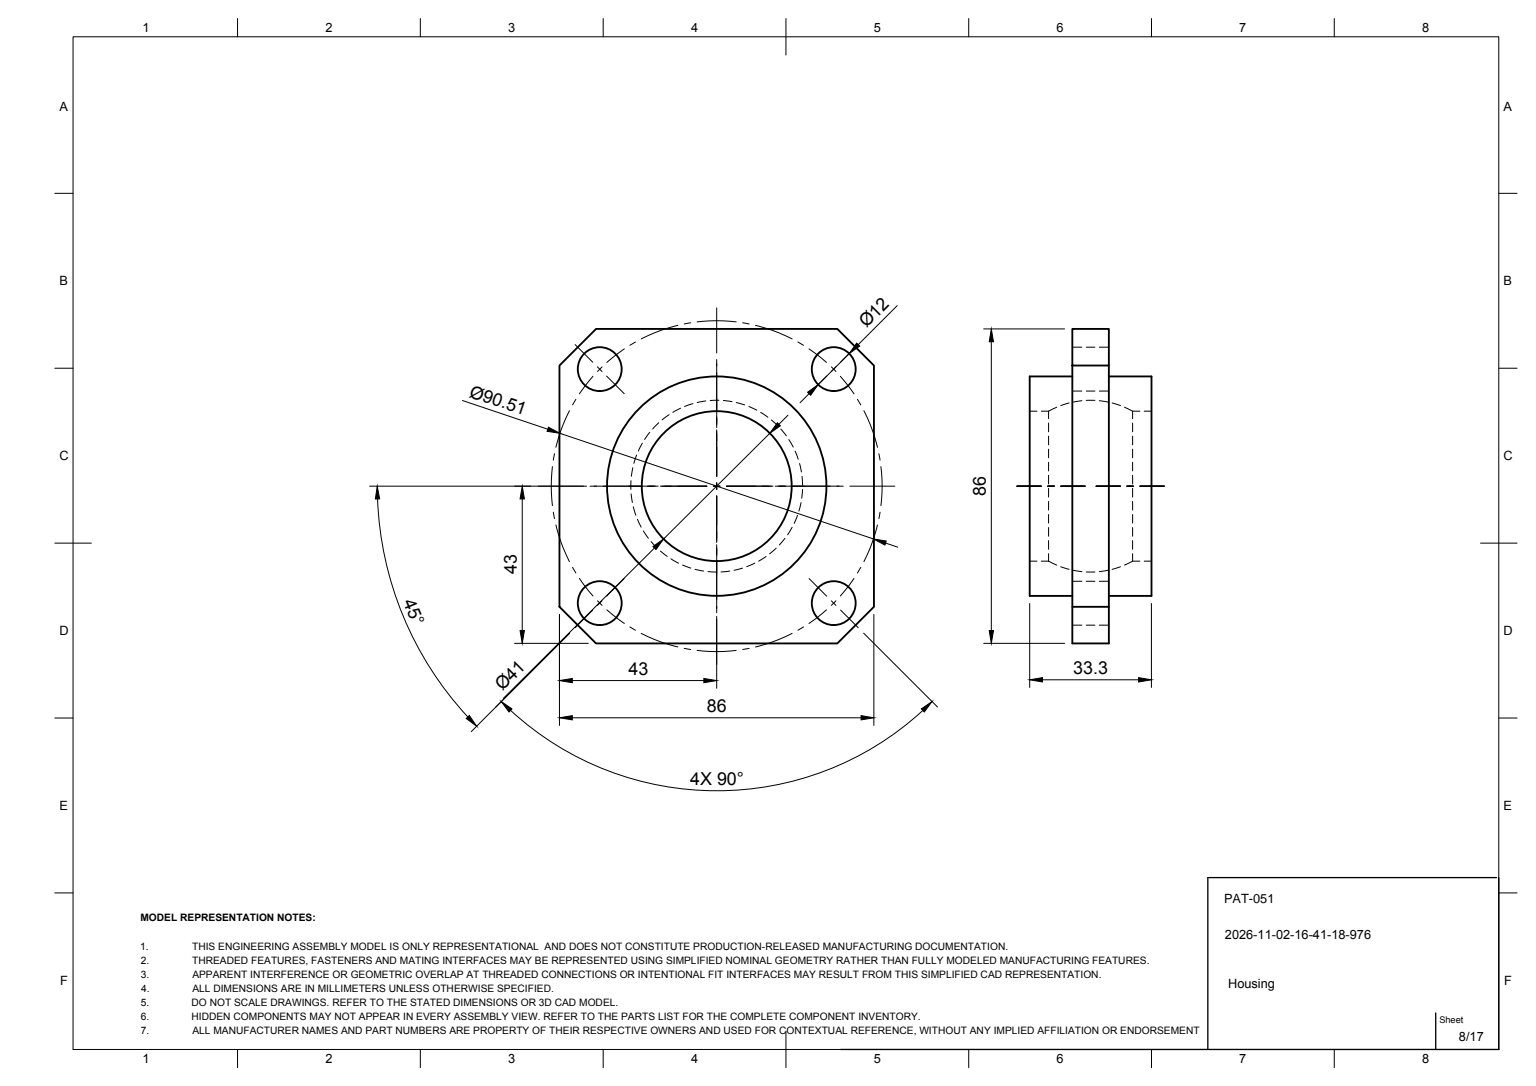
ISO-10303-21;
HEADER;
/* Generated by software containing ST-Developer
 * from STEP Tools, Inc. (www.steptools.com) 
 */

FILE_DESCRIPTION(
/* description */ ('Hand-crank flanged shaft unit'),
/* implementation_level */ '2;1');

FILE_NAME(
/* name */ 'Housing.step',
/* time_stamp */ '2026-10-27T18:35:45-07:00',
/* author */ (''),
/* organization */ (''),
/* preprocessor_version */ 'ST-DEVELOPER v20.2',
/* originating_system */ 'Autodesk Translation Framework v15.17.0.0',
/* authorisation */ '');

FILE_SCHEMA (('AUTOMOTIVE_DESIGN { 1 0 10303 214 3 1 1 }'));
ENDSEC;

DATA;
#10=MECHANICAL_DESIGN_GEOMETRIC_PRESENTATION_REPRESENTATION('',(#288),#6805);
#237=SPHERICAL_SURFACE('',#3681,2.35);
#248=SHAPE_REPRESENTATION_RELATIONSHIP('SRR','None',#6910,#268);
#268=ADVANCED_BREP_SHAPE_REPRESENTATION('',(#309),#6793);
#288=STYLED_ITEM('',(#7070),#309);
#309=MANIFOLD_SOLID_BREP('Body1',#3329);
#358=FACE_BOUND('',#802,.T.);
#359=FACE_BOUND('',#803,.T.);
#360=FACE_BOUND('',#807,.T.);
#361=FACE_BOUND('',#809,.T.);
#362=FACE_BOUND('',#823,.T.);
#363=FACE_BOUND('',#824,.T.);
#364=FACE_BOUND('',#825,.T.);
#365=FACE_BOUND('',#826,.T.);
#366=FACE_BOUND('',#827,.T.);
#367=FACE_BOUND('',#829,.T.);
#368=FACE_BOUND('',#830,.T.);
#369=FACE_BOUND('',#831,.T.);
#370=FACE_BOUND('',#832,.T.);
#371=FACE_BOUND('',#833,.T.);
#442=PLANE('',#3689);
#443=PLANE('',#3690);
#444=PLANE('',#3703);
#445=PLANE('',#3704);
#446=PLANE('',#3705);
#447=PLANE('',#3706);
#448=PLANE('',#3707);
#449=PLANE('',#3708);
#450=PLANE('',#3709);
#451=PLANE('',#3710);
#452=PLANE('',#3711);
#453=PLANE('',#3712);
#573=FACE_OUTER_BOUND('',#799,.T.);
#574=FACE_OUTER_BOUND('',#800,.T.);
#575=FACE_OUTER_BOUND('',#801,.T.);
#576=FACE_OUTER_BOUND('',#804,.T.);
#577=FACE_OUTER_BOUND('',#805,.T.);
#578=FACE_OUTER_BOUND('',#806,.T.);
#579=FACE_OUTER_BOUND('',#808,.T.);
#580=FACE_OUTER_BOUND('',#810,.T.);
#581=FACE_OUTER_BOUND('',#811,.T.);
#582=FACE_OUTER_BOUND('',#812,.T.);
#583=FACE_OUTER_BOUND('',#813,.T.);
#584=FACE_OUTER_BOUND('',#814,.T.);
#585=FACE_OUTER_BOUND('',#815,.T.);
#586=FACE_OUTER_BOUND('',#816,.T.);
#587=FACE_OUTER_BOUND('',#817,.T.);
#588=FACE_OUTER_BOUND('',#818,.T.);
#589=FACE_OUTER_BOUND('',#819,.T.);
#590=FACE_OUTER_BOUND('',#820,.T.);
#591=FACE_OUTER_BOUND('',#821,.T.);
#592=FACE_OUTER_BOUND('',#822,.T.);
#593=FACE_OUTER_BOUND('',#828,.T.);
#799=EDGE_LOOP('',(#2479,#2480,#2481,#2482));
#800=EDGE_LOOP('',(#2483,#2484,#2485,#2486));
#801=EDGE_LOOP('',(#2487,#2488));
#802=EDGE_LOOP('',(#2489));
#803=EDGE_LOOP('',(#2490));
#804=EDGE_LOOP('',(#2491,#2492,#2493,#2494));
#805=EDGE_LOOP('',(#2495,#2496,#2497,#2498));
#806=EDGE_LOOP('',(#2499));
#807=EDGE_LOOP('',(#2500));
#808=EDGE_LOOP('',(#2501));
#809=EDGE_LOOP('',(#2502));
#810=EDGE_LOOP('',(#2503,#2504,#2505,#2506));
#811=EDGE_LOOP('',(#2507,#2508,#2509,#2510));
#812=EDGE_LOOP('',(#2511,#2512,#2513,#2514));
#813=EDGE_LOOP('',(#2515,#2516,#2517,#2518));
#814=EDGE_LOOP('',(#2519,#2520,#2521,#2522));
#815=EDGE_LOOP('',(#2523,#2524,#2525,#2526));
#816=EDGE_LOOP('',(#2527,#2528,#2529,#2530));
#817=EDGE_LOOP('',(#2531,#2532,#2533,#2534));
#818=EDGE_LOOP('',(#2535,#2536,#2537,#2538));
#819=EDGE_LOOP('',(#2539,#2540,#2541,#2542));
#820=EDGE_LOOP('',(#2543,#2544,#2545,#2546));
#821=EDGE_LOOP('',(#2547,#2548,#2549,#2550));
#822=EDGE_LOOP('',(#2551,#2552,#2553,#2554,#2555,#2556,#2557,#2558));
#823=EDGE_LOOP('',(#2559));
#824=EDGE_LOOP('',(#2560));
#825=EDGE_LOOP('',(#2561));
#826=EDGE_LOOP('',(#2562));
#827=EDGE_LOOP('',(#2563));
#828=EDGE_LOOP('',(#2564,#2565,#2566,#2567,#2568,#2569,#2570,#2571));
#829=EDGE_LOOP('',(#2572));
#830=EDGE_LOOP('',(#2573));
#831=EDGE_LOOP('',(#2574));
#832=EDGE_LOOP('',(#2575));
#833=EDGE_LOOP('',(#2576));
#1043=LINE('',#5197,#1271);
#1044=LINE('',#5203,#1272);
#1045=LINE('',#5213,#1273);
#1046=LINE('',#5219,#1274);
#1047=LINE('',#5227,#1275);
#1048=LINE('',#5233,#1276);
#1049=LINE('',#5239,#1277);
#1050=LINE('',#5245,#1278);
#1051=LINE('',#5250,#1279);
#1052=LINE('',#5252,#1280);
#1053=LINE('',#5254,#1281);
#1054=LINE('',#5255,#1282);
#1055=LINE('',#5258,#1283);
#1056=LINE('',#5260,#1284);
#1057=LINE('',#5261,#1285);
#1058=LINE('',#5264,#1286);
#1059=LINE('',#5266,#1287);
#1060=LINE('',#5267,#1288);
#1061=LINE('',#5270,#1289);
#1062=LINE('',#5272,#1290);
#1063=LINE('',#5273,#1291);
#1064=LINE('',#5276,#1292);
#1065=LINE('',#5278,#1293);
#1066=LINE('',#5279,#1294);
#1067=LINE('',#5282,#1295);
#1068=LINE('',#5284,#1296);
#1069=LINE('',#5285,#1297);
#1070=LINE('',#5288,#1298);
#1071=LINE('',#5290,#1299);
#1072=LINE('',#5291,#1300);
#1073=LINE('',#5293,#1301);
#1074=LINE('',#5294,#1302);
#1271=VECTOR('',#4248,2.05);
#1272=VECTOR('',#4255,2.05);
#1273=VECTOR('',#4266,3.);
#1274=VECTOR('',#4273,3.);
#1275=VECTOR('',#4284,0.6);
#1276=VECTOR('',#4291,0.6);
#1277=VECTOR('',#4298,0.6);
#1278=VECTOR('',#4305,0.6);
#1279=VECTOR('',#4310,1.);
#1280=VECTOR('',#4311,1.);
#1281=VECTOR('',#4312,1.);
#1282=VECTOR('',#4313,1.);
#1283=VECTOR('',#4316,1.);
#1284=VECTOR('',#4317,1.);
#1285=VECTOR('',#4318,1.);
#1286=VECTOR('',#4321,1.);
#1287=VECTOR('',#4322,1.);
#1288=VECTOR('',#4323,1.);
#1289=VECTOR('',#4326,1.);
#1290=VECTOR('',#4327,1.);
#1291=VECTOR('',#4328,1.);
#1292=VECTOR('',#4331,1.);
#1293=VECTOR('',#4332,1.);
#1294=VECTOR('',#4333,1.);
#1295=VECTOR('',#4336,1.);
#1296=VECTOR('',#4337,1.);
#1297=VECTOR('',#4338,1.);
#1298=VECTOR('',#4341,1.);
#1299=VECTOR('',#4342,1.);
#1300=VECTOR('',#4343,1.);
#1301=VECTOR('',#4346,1.);
#1302=VECTOR('',#4347,1.);
#1489=CIRCLE('',#3676,2.05);
#1490=CIRCLE('',#3677,2.05);
#1491=CIRCLE('',#3679,2.05);
#1492=CIRCLE('',#3680,2.05);
#1493=CIRCLE('',#3682,2.35);
#1494=CIRCLE('',#3684,3.);
#1495=CIRCLE('',#3685,3.);
#1496=CIRCLE('',#3687,3.);
#1497=CIRCLE('',#3688,3.);
#1498=CIRCLE('',#3692,0.6);
#1499=CIRCLE('',#3693,0.6);
#1500=CIRCLE('',#3695,0.6);
#1501=CIRCLE('',#3696,0.6);
#1502=CIRCLE('',#3698,0.6);
#1503=CIRCLE('',#3699,0.6);
#1504=CIRCLE('',#3701,0.6);
#1505=CIRCLE('',#3702,0.6);
#1645=VERTEX_POINT('',#5194);
#1646=VERTEX_POINT('',#5196);
#1647=VERTEX_POINT('',#5200);
#1648=VERTEX_POINT('',#5202);
#1649=VERTEX_POINT('',#5206);
#1650=VERTEX_POINT('',#5207);
#1651=VERTEX_POINT('',#5210);
#1652=VERTEX_POINT('',#5212);
#1653=VERTEX_POINT('',#5216);
#1654=VERTEX_POINT('',#5218);
#1655=VERTEX_POINT('',#5224);
#1656=VERTEX_POINT('',#5226);
#1657=VERTEX_POINT('',#5230);
#1658=VERTEX_POINT('',#5232);
#1659=VERTEX_POINT('',#5236);
#1660=VERTEX_POINT('',#5238);
#1661=VERTEX_POINT('',#5242);
#1662=VERTEX_POINT('',#5244);
#1663=VERTEX_POINT('',#5248);
#1664=VERTEX_POINT('',#5249);
#1665=VERTEX_POINT('',#5251);
#1666=VERTEX_POINT('',#5253);
#1667=VERTEX_POINT('',#5257);
#1668=VERTEX_POINT('',#5259);
#1669=VERTEX_POINT('',#5263);
#1670=VERTEX_POINT('',#5265);
#1671=VERTEX_POINT('',#5269);
#1672=VERTEX_POINT('',#5271);
#1673=VERTEX_POINT('',#5275);
#1674=VERTEX_POINT('',#5277);
#1675=VERTEX_POINT('',#5281);
#1676=VERTEX_POINT('',#5283);
#1677=VERTEX_POINT('',#5287);
#1678=VERTEX_POINT('',#5289);
#1957=EDGE_CURVE('',#1645,#1645,#1489,.T.);
#1958=EDGE_CURVE('',#1645,#1646,#1043,.T.);
#1959=EDGE_CURVE('',#1646,#1646,#1490,.T.);
#1960=EDGE_CURVE('',#1647,#1647,#1491,.T.);
#1961=EDGE_CURVE('',#1647,#1648,#1044,.T.);
#1962=EDGE_CURVE('',#1648,#1648,#1492,.T.);
#1963=EDGE_CURVE('',#1649,#1650,#1493,.T.);
#1964=EDGE_CURVE('',#1651,#1651,#1494,.T.);
#1965=EDGE_CURVE('',#1651,#1652,#1045,.T.);
#1966=EDGE_CURVE('',#1652,#1652,#1495,.T.);
#1967=EDGE_CURVE('',#1653,#1653,#1496,.T.);
#1968=EDGE_CURVE('',#1653,#1654,#1046,.T.);
#1969=EDGE_CURVE('',#1654,#1654,#1497,.T.);
#1970=EDGE_CURVE('',#1655,#1655,#1498,.T.);
#1971=EDGE_CURVE('',#1655,#1656,#1047,.T.);
#1972=EDGE_CURVE('',#1656,#1656,#1499,.T.);
#1973=EDGE_CURVE('',#1657,#1657,#1500,.T.);
#1974=EDGE_CURVE('',#1657,#1658,#1048,.T.);
#1975=EDGE_CURVE('',#1658,#1658,#1501,.T.);
#1976=EDGE_CURVE('',#1659,#1659,#1502,.T.);
#1977=EDGE_CURVE('',#1659,#1660,#1049,.T.);
#1978=EDGE_CURVE('',#1660,#1660,#1503,.T.);
#1979=EDGE_CURVE('',#1661,#1661,#1504,.T.);
#1980=EDGE_CURVE('',#1661,#1662,#1050,.T.);
#1981=EDGE_CURVE('',#1662,#1662,#1505,.T.);
#1982=EDGE_CURVE('',#1663,#1664,#1051,.T.);
#1983=EDGE_CURVE('',#1664,#1665,#1052,.T.);
#1984=EDGE_CURVE('',#1666,#1665,#1053,.T.);
#1985=EDGE_CURVE('',#1663,#1666,#1054,.T.);
#1986=EDGE_CURVE('',#1667,#1663,#1055,.T.);
#1987=EDGE_CURVE('',#1668,#1666,#1056,.T.);
#1988=EDGE_CURVE('',#1667,#1668,#1057,.T.);
#1989=EDGE_CURVE('',#1669,#1667,#1058,.T.);
#1990=EDGE_CURVE('',#1670,#1668,#1059,.T.);
#1991=EDGE_CURVE('',#1669,#1670,#1060,.T.);
#1992=EDGE_CURVE('',#1671,#1669,#1061,.T.);
#1993=EDGE_CURVE('',#1672,#1670,#1062,.T.);
#1994=EDGE_CURVE('',#1671,#1672,#1063,.T.);
#1995=EDGE_CURVE('',#1673,#1671,#1064,.T.);
#1996=EDGE_CURVE('',#1674,#1672,#1065,.T.);
#1997=EDGE_CURVE('',#1673,#1674,#1066,.T.);
#1998=EDGE_CURVE('',#1675,#1673,#1067,.T.);
#1999=EDGE_CURVE('',#1676,#1674,#1068,.T.);
#2000=EDGE_CURVE('',#1675,#1676,#1069,.T.);
#2001=EDGE_CURVE('',#1677,#1675,#1070,.T.);
#2002=EDGE_CURVE('',#1678,#1676,#1071,.T.);
#2003=EDGE_CURVE('',#1677,#1678,#1072,.T.);
#2004=EDGE_CURVE('',#1664,#1677,#1073,.T.);
#2005=EDGE_CURVE('',#1665,#1678,#1074,.T.);
#2479=ORIENTED_EDGE('',*,*,#1957,.F.);
#2480=ORIENTED_EDGE('',*,*,#1958,.T.);
#2481=ORIENTED_EDGE('',*,*,#1959,.F.);
#2482=ORIENTED_EDGE('',*,*,#1958,.F.);
#2483=ORIENTED_EDGE('',*,*,#1960,.F.);
#2484=ORIENTED_EDGE('',*,*,#1961,.T.);
#2485=ORIENTED_EDGE('',*,*,#1962,.F.);
#2486=ORIENTED_EDGE('',*,*,#1961,.F.);
#2487=ORIENTED_EDGE('',*,*,#1963,.T.);
#2488=ORIENTED_EDGE('',*,*,#1963,.F.);
#2489=ORIENTED_EDGE('',*,*,#1960,.T.);
#2490=ORIENTED_EDGE('',*,*,#1959,.T.);
#2491=ORIENTED_EDGE('',*,*,#1964,.F.);
#2492=ORIENTED_EDGE('',*,*,#1965,.T.);
#2493=ORIENTED_EDGE('',*,*,#1966,.F.);
#2494=ORIENTED_EDGE('',*,*,#1965,.F.);
#2495=ORIENTED_EDGE('',*,*,#1967,.F.);
#2496=ORIENTED_EDGE('',*,*,#1968,.T.);
#2497=ORIENTED_EDGE('',*,*,#1969,.F.);
#2498=ORIENTED_EDGE('',*,*,#1968,.F.);
#2499=ORIENTED_EDGE('',*,*,#1966,.T.);
#2500=ORIENTED_EDGE('',*,*,#1957,.T.);
#2501=ORIENTED_EDGE('',*,*,#1967,.T.);
#2502=ORIENTED_EDGE('',*,*,#1962,.T.);
#2503=ORIENTED_EDGE('',*,*,#1970,.F.);
#2504=ORIENTED_EDGE('',*,*,#1971,.T.);
#2505=ORIENTED_EDGE('',*,*,#1972,.F.);
#2506=ORIENTED_EDGE('',*,*,#1971,.F.);
#2507=ORIENTED_EDGE('',*,*,#1973,.F.);
#2508=ORIENTED_EDGE('',*,*,#1974,.T.);
#2509=ORIENTED_EDGE('',*,*,#1975,.F.);
#2510=ORIENTED_EDGE('',*,*,#1974,.F.);
#2511=ORIENTED_EDGE('',*,*,#1976,.F.);
#2512=ORIENTED_EDGE('',*,*,#1977,.T.);
#2513=ORIENTED_EDGE('',*,*,#1978,.F.);
#2514=ORIENTED_EDGE('',*,*,#1977,.F.);
#2515=ORIENTED_EDGE('',*,*,#1979,.F.);
#2516=ORIENTED_EDGE('',*,*,#1980,.T.);
#2517=ORIENTED_EDGE('',*,*,#1981,.F.);
#2518=ORIENTED_EDGE('',*,*,#1980,.F.);
#2519=ORIENTED_EDGE('',*,*,#1982,.T.);
#2520=ORIENTED_EDGE('',*,*,#1983,.T.);
#2521=ORIENTED_EDGE('',*,*,#1984,.F.);
#2522=ORIENTED_EDGE('',*,*,#1985,.F.);
#2523=ORIENTED_EDGE('',*,*,#1986,.T.);
#2524=ORIENTED_EDGE('',*,*,#1985,.T.);
#2525=ORIENTED_EDGE('',*,*,#1987,.F.);
#2526=ORIENTED_EDGE('',*,*,#1988,.F.);
#2527=ORIENTED_EDGE('',*,*,#1989,.T.);
#2528=ORIENTED_EDGE('',*,*,#1988,.T.);
#2529=ORIENTED_EDGE('',*,*,#1990,.F.);
#2530=ORIENTED_EDGE('',*,*,#1991,.F.);
#2531=ORIENTED_EDGE('',*,*,#1992,.T.);
#2532=ORIENTED_EDGE('',*,*,#1991,.T.);
#2533=ORIENTED_EDGE('',*,*,#1993,.F.);
#2534=ORIENTED_EDGE('',*,*,#1994,.F.);
#2535=ORIENTED_EDGE('',*,*,#1995,.T.);
#2536=ORIENTED_EDGE('',*,*,#1994,.T.);
#2537=ORIENTED_EDGE('',*,*,#1996,.F.);
#2538=ORIENTED_EDGE('',*,*,#1997,.F.);
#2539=ORIENTED_EDGE('',*,*,#1998,.T.);
#2540=ORIENTED_EDGE('',*,*,#1997,.T.);
#2541=ORIENTED_EDGE('',*,*,#1999,.F.);
#2542=ORIENTED_EDGE('',*,*,#2000,.F.);
#2543=ORIENTED_EDGE('',*,*,#2001,.T.);
#2544=ORIENTED_EDGE('',*,*,#2000,.T.);
#2545=ORIENTED_EDGE('',*,*,#2002,.F.);
#2546=ORIENTED_EDGE('',*,*,#2003,.F.);
#2547=ORIENTED_EDGE('',*,*,#2004,.T.);
#2548=ORIENTED_EDGE('',*,*,#2003,.T.);
#2549=ORIENTED_EDGE('',*,*,#2005,.F.);
#2550=ORIENTED_EDGE('',*,*,#1983,.F.);
#2551=ORIENTED_EDGE('',*,*,#2005,.T.);
#2552=ORIENTED_EDGE('',*,*,#2002,.T.);
#2553=ORIENTED_EDGE('',*,*,#1999,.T.);
#2554=ORIENTED_EDGE('',*,*,#1996,.T.);
#2555=ORIENTED_EDGE('',*,*,#1993,.T.);
#2556=ORIENTED_EDGE('',*,*,#1990,.T.);
#2557=ORIENTED_EDGE('',*,*,#1987,.T.);
#2558=ORIENTED_EDGE('',*,*,#1984,.T.);
#2559=ORIENTED_EDGE('',*,*,#1969,.T.);
#2560=ORIENTED_EDGE('',*,*,#1972,.T.);
#2561=ORIENTED_EDGE('',*,*,#1975,.T.);
#2562=ORIENTED_EDGE('',*,*,#1978,.T.);
#2563=ORIENTED_EDGE('',*,*,#1981,.T.);
#2564=ORIENTED_EDGE('',*,*,#2004,.F.);
#2565=ORIENTED_EDGE('',*,*,#1982,.F.);
#2566=ORIENTED_EDGE('',*,*,#1986,.F.);
#2567=ORIENTED_EDGE('',*,*,#1989,.F.);
#2568=ORIENTED_EDGE('',*,*,#1992,.F.);
#2569=ORIENTED_EDGE('',*,*,#1995,.F.);
#2570=ORIENTED_EDGE('',*,*,#1998,.F.);
#2571=ORIENTED_EDGE('',*,*,#2001,.F.);
#2572=ORIENTED_EDGE('',*,*,#1964,.T.);
#2573=ORIENTED_EDGE('',*,*,#1970,.T.);
#2574=ORIENTED_EDGE('',*,*,#1973,.T.);
#2575=ORIENTED_EDGE('',*,*,#1976,.T.);
#2576=ORIENTED_EDGE('',*,*,#1979,.T.);
#3093=CYLINDRICAL_SURFACE('',#3675,2.05);
#3094=CYLINDRICAL_SURFACE('',#3678,2.05);
#3095=CYLINDRICAL_SURFACE('',#3683,3.);
#3096=CYLINDRICAL_SURFACE('',#3686,3.);
#3097=CYLINDRICAL_SURFACE('',#3691,0.6);
#3098=CYLINDRICAL_SURFACE('',#3694,0.6);
#3099=CYLINDRICAL_SURFACE('',#3697,0.6);
#3100=CYLINDRICAL_SURFACE('',#3700,0.6);
#3190=ADVANCED_FACE('',(#573),#3093,.F.);
#3191=ADVANCED_FACE('',(#574),#3094,.F.);
#3192=ADVANCED_FACE('',(#575,#358,#359),#237,.F.);
#3193=ADVANCED_FACE('',(#576),#3095,.T.);
#3194=ADVANCED_FACE('',(#577),#3096,.T.);
#3195=ADVANCED_FACE('',(#578,#360),#442,.F.);
#3196=ADVANCED_FACE('',(#579,#361),#443,.T.);
#3197=ADVANCED_FACE('',(#580),#3097,.F.);
#3198=ADVANCED_FACE('',(#581),#3098,.F.);
#3199=ADVANCED_FACE('',(#582),#3099,.F.);
#3200=ADVANCED_FACE('',(#583),#3100,.F.);
#3201=ADVANCED_FACE('',(#584),#444,.T.);
#3202=ADVANCED_FACE('',(#585),#445,.T.);
#3203=ADVANCED_FACE('',(#586),#446,.T.);
#3204=ADVANCED_FACE('',(#587),#447,.T.);
#3205=ADVANCED_FACE('',(#588),#448,.T.);
#3206=ADVANCED_FACE('',(#589),#449,.T.);
#3207=ADVANCED_FACE('',(#590),#450,.T.);
#3208=ADVANCED_FACE('',(#591),#451,.T.);
#3209=ADVANCED_FACE('',(#592,#362,#363,#364,#365,#366),#452,.T.);
#3210=ADVANCED_FACE('',(#593,#367,#368,#369,#370,#371),#453,.F.);
#3329=CLOSED_SHELL('',(#3190,#3191,#3192,#3193,#3194,#3195,#3196,#3197,
#3198,#3199,#3200,#3201,#3202,#3203,#3204,#3205,#3206,#3207,#3208,#3209,
#3210));
#3674=AXIS2_PLACEMENT_3D('',#5192,#4242,#4243);
#3675=AXIS2_PLACEMENT_3D('',#5193,#4244,#4245);
#3676=AXIS2_PLACEMENT_3D('',#5195,#4246,#4247);
#3677=AXIS2_PLACEMENT_3D('',#5198,#4249,#4250);
#3678=AXIS2_PLACEMENT_3D('',#5199,#4251,#4252);
#3679=AXIS2_PLACEMENT_3D('',#5201,#4253,#4254);
#3680=AXIS2_PLACEMENT_3D('',#5204,#4256,#4257);
#3681=AXIS2_PLACEMENT_3D('',#5205,#4258,#4259);
#3682=AXIS2_PLACEMENT_3D('',#5208,#4260,#4261);
#3683=AXIS2_PLACEMENT_3D('',#5209,#4262,#4263);
#3684=AXIS2_PLACEMENT_3D('',#5211,#4264,#4265);
#3685=AXIS2_PLACEMENT_3D('',#5214,#4267,#4268);
#3686=AXIS2_PLACEMENT_3D('',#5215,#4269,#4270);
#3687=AXIS2_PLACEMENT_3D('',#5217,#4271,#4272);
#3688=AXIS2_PLACEMENT_3D('',#5220,#4274,#4275);
#3689=AXIS2_PLACEMENT_3D('',#5221,#4276,#4277);
#3690=AXIS2_PLACEMENT_3D('',#5222,#4278,#4279);
#3691=AXIS2_PLACEMENT_3D('',#5223,#4280,#4281);
#3692=AXIS2_PLACEMENT_3D('',#5225,#4282,#4283);
#3693=AXIS2_PLACEMENT_3D('',#5228,#4285,#4286);
#3694=AXIS2_PLACEMENT_3D('',#5229,#4287,#4288);
#3695=AXIS2_PLACEMENT_3D('',#5231,#4289,#4290);
#3696=AXIS2_PLACEMENT_3D('',#5234,#4292,#4293);
#3697=AXIS2_PLACEMENT_3D('',#5235,#4294,#4295);
#3698=AXIS2_PLACEMENT_3D('',#5237,#4296,#4297);
#3699=AXIS2_PLACEMENT_3D('',#5240,#4299,#4300);
#3700=AXIS2_PLACEMENT_3D('',#5241,#4301,#4302);
#3701=AXIS2_PLACEMENT_3D('',#5243,#4303,#4304);
#3702=AXIS2_PLACEMENT_3D('',#5246,#4306,#4307);
#3703=AXIS2_PLACEMENT_3D('',#5247,#4308,#4309);
#3704=AXIS2_PLACEMENT_3D('',#5256,#4314,#4315);
#3705=AXIS2_PLACEMENT_3D('',#5262,#4319,#4320);
#3706=AXIS2_PLACEMENT_3D('',#5268,#4324,#4325);
#3707=AXIS2_PLACEMENT_3D('',#5274,#4329,#4330);
#3708=AXIS2_PLACEMENT_3D('',#5280,#4334,#4335);
#3709=AXIS2_PLACEMENT_3D('',#5286,#4339,#4340);
#3710=AXIS2_PLACEMENT_3D('',#5292,#4344,#4345);
#3711=AXIS2_PLACEMENT_3D('',#5295,#4348,#4349);
#3712=AXIS2_PLACEMENT_3D('',#5296,#4350,#4351);
#4242=DIRECTION('axis',(0.,0.,1.));
#4243=DIRECTION('refdir',(1.,0.,0.));
#4244=DIRECTION('center_axis',(0.,1.,0.));
#4245=DIRECTION('ref_axis',(1.,0.,0.));
#4246=DIRECTION('center_axis',(0.,1.,0.));
#4247=DIRECTION('ref_axis',(1.,0.,0.));
#4248=DIRECTION('',(0.,1.,0.));
#4249=DIRECTION('center_axis',(0.,-1.,0.));
#4250=DIRECTION('ref_axis',(1.,0.,0.));
#4251=DIRECTION('center_axis',(0.,1.,0.));
#4252=DIRECTION('ref_axis',(1.,0.,0.));
#4253=DIRECTION('center_axis',(0.,1.,0.));
#4254=DIRECTION('ref_axis',(1.,0.,0.));
#4255=DIRECTION('',(0.,1.,0.));
#4256=DIRECTION('center_axis',(0.,-1.,0.));
#4257=DIRECTION('ref_axis',(1.,0.,0.));
#4258=DIRECTION('center_axis',(6.12323399573677E-17,0.,1.));
#4259=DIRECTION('ref_axis',(1.,0.,0.));
#4260=DIRECTION('center_axis',(-1.22464679914735E-16,1.,0.));
#4261=DIRECTION('ref_axis',(-1.,-1.22464679914735E-16,0.));
#4262=DIRECTION('center_axis',(0.,1.,0.));
#4263=DIRECTION('ref_axis',(1.,0.,0.));
#4264=DIRECTION('center_axis',(0.,1.,0.));
#4265=DIRECTION('ref_axis',(1.,0.,0.));
#4266=DIRECTION('',(0.,-1.,0.));
#4267=DIRECTION('center_axis',(0.,-1.,0.));
#4268=DIRECTION('ref_axis',(1.,0.,0.));
#4269=DIRECTION('center_axis',(0.,1.,0.));
#4270=DIRECTION('ref_axis',(1.,0.,0.));
#4271=DIRECTION('center_axis',(0.,1.,0.));
#4272=DIRECTION('ref_axis',(1.,0.,0.));
#4273=DIRECTION('',(0.,-1.,0.));
#4274=DIRECTION('center_axis',(0.,-1.,0.));
#4275=DIRECTION('ref_axis',(1.,0.,0.));
#4276=DIRECTION('center_axis',(0.,1.,0.));
#4277=DIRECTION('ref_axis',(1.,0.,0.));
#4278=DIRECTION('center_axis',(0.,1.,0.));
#4279=DIRECTION('ref_axis',(1.,0.,0.));
#4280=DIRECTION('center_axis',(0.,1.,0.));
#4281=DIRECTION('ref_axis',(1.,0.,0.));
#4282=DIRECTION('center_axis',(0.,1.,0.));
#4283=DIRECTION('ref_axis',(1.,0.,0.));
#4284=DIRECTION('',(0.,1.,0.));
#4285=DIRECTION('center_axis',(0.,-1.,0.));
#4286=DIRECTION('ref_axis',(1.,0.,0.));
#4287=DIRECTION('center_axis',(0.,1.,0.));
#4288=DIRECTION('ref_axis',(1.,0.,0.));
#4289=DIRECTION('center_axis',(0.,1.,0.));
#4290=DIRECTION('ref_axis',(1.,0.,0.));
#4291=DIRECTION('',(0.,1.,0.));
#4292=DIRECTION('center_axis',(0.,-1.,0.));
#4293=DIRECTION('ref_axis',(1.,0.,0.));
#4294=DIRECTION('center_axis',(0.,1.,0.));
#4295=DIRECTION('ref_axis',(1.,0.,0.));
#4296=DIRECTION('center_axis',(0.,1.,0.));
#4297=DIRECTION('ref_axis',(1.,0.,0.));
#4298=DIRECTION('',(0.,1.,0.));
#4299=DIRECTION('center_axis',(0.,-1.,0.));
#4300=DIRECTION('ref_axis',(1.,0.,0.));
#4301=DIRECTION('center_axis',(0.,1.,0.));
#4302=DIRECTION('ref_axis',(1.,0.,0.));
#4303=DIRECTION('center_axis',(0.,1.,0.));
#4304=DIRECTION('ref_axis',(1.,0.,0.));
#4305=DIRECTION('',(0.,1.,0.));
#4306=DIRECTION('center_axis',(0.,-1.,0.));
#4307=DIRECTION('ref_axis',(1.,0.,0.));
#4308=DIRECTION('center_axis',(-1.,0.,0.));
#4309=DIRECTION('ref_axis',(0.,0.,1.));
#4310=DIRECTION('',(0.,0.,1.));
#4311=DIRECTION('',(0.,1.,0.));
#4312=DIRECTION('',(0.,0.,1.));
#4313=DIRECTION('',(0.,1.,0.));
#4314=DIRECTION('center_axis',(-0.707106781186548,0.,-0.707106781186548));
#4315=DIRECTION('ref_axis',(-0.707106781186548,0.,0.707106781186548));
#4316=DIRECTION('',(-0.707106781186548,0.,0.707106781186548));
#4317=DIRECTION('',(-0.707106781186548,0.,0.707106781186548));
#4318=DIRECTION('',(0.,1.,0.));
#4319=DIRECTION('center_axis',(0.,0.,-1.));
#4320=DIRECTION('ref_axis',(-1.,0.,0.));
#4321=DIRECTION('',(-1.,0.,0.));
#4322=DIRECTION('',(-1.,0.,0.));
#4323=DIRECTION('',(0.,1.,0.));
#4324=DIRECTION('center_axis',(0.707106781186548,0.,-0.707106781186548));
#4325=DIRECTION('ref_axis',(-0.707106781186548,0.,-0.707106781186548));
#4326=DIRECTION('',(-0.707106781186548,0.,-0.707106781186548));
#4327=DIRECTION('',(-0.707106781186548,0.,-0.707106781186548));
#4328=DIRECTION('',(0.,1.,0.));
#4329=DIRECTION('center_axis',(1.,0.,0.));
#4330=DIRECTION('ref_axis',(0.,0.,-1.));
#4331=DIRECTION('',(0.,0.,-1.));
#4332=DIRECTION('',(0.,0.,-1.));
#4333=DIRECTION('',(0.,1.,0.));
#4334=DIRECTION('center_axis',(0.707106781186548,0.,0.707106781186548));
#4335=DIRECTION('ref_axis',(0.707106781186548,0.,-0.707106781186548));
#4336=DIRECTION('',(0.707106781186548,0.,-0.707106781186548));
#4337=DIRECTION('',(0.707106781186548,0.,-0.707106781186548));
#4338=DIRECTION('',(0.,1.,0.));
#4339=DIRECTION('center_axis',(0.,0.,1.));
#4340=DIRECTION('ref_axis',(1.,0.,0.));
#4341=DIRECTION('',(1.,0.,0.));
#4342=DIRECTION('',(1.,0.,0.));
#4343=DIRECTION('',(0.,1.,0.));
#4344=DIRECTION('center_axis',(-0.707106781186548,0.,0.707106781186548));
#4345=DIRECTION('ref_axis',(0.707106781186548,0.,0.707106781186548));
#4346=DIRECTION('',(0.707106781186548,0.,0.707106781186548));
#4347=DIRECTION('',(0.707106781186548,0.,0.707106781186548));
#4348=DIRECTION('center_axis',(0.,1.,0.));
#4349=DIRECTION('ref_axis',(0.,0.,1.));
#4350=DIRECTION('center_axis',(0.,1.,0.));
#4351=DIRECTION('ref_axis',(1.,0.,0.));
#5192=CARTESIAN_POINT('',(0.,0.,0.));
#5193=CARTESIAN_POINT('Origin',(0.,0.,0.));
#5194=CARTESIAN_POINT('',(-2.05,-1.665,2.51052593825207E-16));
#5195=CARTESIAN_POINT('Origin',(0.,-1.665,0.));
#5196=CARTESIAN_POINT('',(-2.05,-1.14891252930761,-2.51052593825207E-16));
#5197=CARTESIAN_POINT('',(-2.05,0.,2.51052593825207E-16));
#5198=CARTESIAN_POINT('Origin',(0.,-1.14891252930761,0.));
#5199=CARTESIAN_POINT('Origin',(0.,0.,0.));
#5200=CARTESIAN_POINT('',(-2.05,1.14891252930761,2.51052593825207E-16));
#5201=CARTESIAN_POINT('Origin',(0.,1.14891252930761,0.));
#5202=CARTESIAN_POINT('',(-2.05,1.665,-2.51052593825207E-16));
#5203=CARTESIAN_POINT('',(-2.05,0.,2.51052593825207E-16));
#5204=CARTESIAN_POINT('Origin',(0.,1.665,0.));
#5205=CARTESIAN_POINT('Origin',(0.,0.,0.));
#5206=CARTESIAN_POINT('',(-1.43895998899814E-16,-1.76221774462768E-32,-2.35));
#5207=CARTESIAN_POINT('',(-1.43895998899814E-16,-1.76221774462768E-32,2.35));
#5208=CARTESIAN_POINT('Origin',(0.,0.,0.));
#5209=CARTESIAN_POINT('Origin',(0.,0.,0.));
#5210=CARTESIAN_POINT('',(-3.,-0.5,3.67394039744206E-16));
#5211=CARTESIAN_POINT('Origin',(0.,-0.5,0.));
#5212=CARTESIAN_POINT('',(-3.,-1.665,3.67394039744206E-16));
#5213=CARTESIAN_POINT('',(-3.,0.,3.67394039744206E-16));
#5214=CARTESIAN_POINT('Origin',(0.,-1.665,0.));
#5215=CARTESIAN_POINT('Origin',(0.,0.,0.));
#5216=CARTESIAN_POINT('',(-3.,1.665,3.67394039744206E-16));
#5217=CARTESIAN_POINT('Origin',(0.,1.665,0.));
#5218=CARTESIAN_POINT('',(-3.,0.5,-3.67394039744206E-16));
#5219=CARTESIAN_POINT('',(-3.,0.,3.67394039744206E-16));
#5220=CARTESIAN_POINT('Origin',(0.,0.5,0.));
#5221=CARTESIAN_POINT('Origin',(0.,-1.665,0.));
#5222=CARTESIAN_POINT('Origin',(0.,1.665,0.));
#5223=CARTESIAN_POINT('Origin',(3.2,0.,3.2));
#5224=CARTESIAN_POINT('',(2.6,-0.5,3.2));
#5225=CARTESIAN_POINT('Origin',(3.2,-0.5,3.2));
#5226=CARTESIAN_POINT('',(2.6,0.5,3.2));
#5227=CARTESIAN_POINT('',(2.6,0.,3.2));
#5228=CARTESIAN_POINT('Origin',(3.2,0.5,3.2));
#5229=CARTESIAN_POINT('Origin',(-3.2,0.,-3.2));
#5230=CARTESIAN_POINT('',(-3.8,-0.5,-3.2));
#5231=CARTESIAN_POINT('Origin',(-3.2,-0.5,-3.2));
#5232=CARTESIAN_POINT('',(-3.8,0.5,-3.2));
#5233=CARTESIAN_POINT('',(-3.8,0.,-3.2));
#5234=CARTESIAN_POINT('Origin',(-3.2,0.5,-3.2));
#5235=CARTESIAN_POINT('Origin',(-3.2,0.,3.2));
#5236=CARTESIAN_POINT('',(-3.8,-0.5,3.2));
#5237=CARTESIAN_POINT('Origin',(-3.2,-0.5,3.2));
#5238=CARTESIAN_POINT('',(-3.8,0.5,3.2));
#5239=CARTESIAN_POINT('',(-3.8,0.,3.2));
#5240=CARTESIAN_POINT('Origin',(-3.2,0.5,3.2));
#5241=CARTESIAN_POINT('Origin',(3.2,0.,-3.2));
#5242=CARTESIAN_POINT('',(2.6,-0.5,-3.2));
#5243=CARTESIAN_POINT('Origin',(3.2,-0.5,-3.2));
#5244=CARTESIAN_POINT('',(2.6,0.5,-3.2));
#5245=CARTESIAN_POINT('',(2.6,0.,-3.2));
#5246=CARTESIAN_POINT('Origin',(3.2,0.5,-3.2));
#5247=CARTESIAN_POINT('Origin',(-4.3,-0.5,-3.3));
#5248=CARTESIAN_POINT('',(-4.3,-0.5,-3.3));
#5249=CARTESIAN_POINT('',(-4.3,-0.5,3.3));
#5250=CARTESIAN_POINT('',(-4.3,-0.5,-3.3));
#5251=CARTESIAN_POINT('',(-4.3,0.5,3.3));
#5252=CARTESIAN_POINT('',(-4.3,-0.5,3.3));
#5253=CARTESIAN_POINT('',(-4.3,0.5,-3.3));
#5254=CARTESIAN_POINT('',(-4.3,0.5,-3.3));
#5255=CARTESIAN_POINT('',(-4.3,-0.5,-3.3));
#5256=CARTESIAN_POINT('Origin',(-3.3,-0.5,-4.3));
#5257=CARTESIAN_POINT('',(-3.3,-0.5,-4.3));
#5258=CARTESIAN_POINT('',(-3.3,-0.5,-4.3));
#5259=CARTESIAN_POINT('',(-3.3,0.5,-4.3));
#5260=CARTESIAN_POINT('',(-3.3,0.5,-4.3));
#5261=CARTESIAN_POINT('',(-3.3,-0.5,-4.3));
#5262=CARTESIAN_POINT('Origin',(3.3,-0.5,-4.3));
#5263=CARTESIAN_POINT('',(3.3,-0.5,-4.3));
#5264=CARTESIAN_POINT('',(3.3,-0.5,-4.3));
#5265=CARTESIAN_POINT('',(3.3,0.5,-4.3));
#5266=CARTESIAN_POINT('',(3.3,0.5,-4.3));
#5267=CARTESIAN_POINT('',(3.3,-0.5,-4.3));
#5268=CARTESIAN_POINT('Origin',(4.3,-0.5,-3.3));
#5269=CARTESIAN_POINT('',(4.3,-0.5,-3.3));
#5270=CARTESIAN_POINT('',(4.3,-0.5,-3.3));
#5271=CARTESIAN_POINT('',(4.3,0.5,-3.3));
#5272=CARTESIAN_POINT('',(4.3,0.5,-3.3));
#5273=CARTESIAN_POINT('',(4.3,-0.5,-3.3));
#5274=CARTESIAN_POINT('Origin',(4.3,-0.5,3.3));
#5275=CARTESIAN_POINT('',(4.3,-0.5,3.3));
#5276=CARTESIAN_POINT('',(4.3,-0.5,3.3));
#5277=CARTESIAN_POINT('',(4.3,0.5,3.3));
#5278=CARTESIAN_POINT('',(4.3,0.5,3.3));
#5279=CARTESIAN_POINT('',(4.3,-0.5,3.3));
#5280=CARTESIAN_POINT('Origin',(3.3,-0.5,4.3));
#5281=CARTESIAN_POINT('',(3.3,-0.5,4.3));
#5282=CARTESIAN_POINT('',(3.3,-0.5,4.3));
#5283=CARTESIAN_POINT('',(3.3,0.5,4.3));
#5284=CARTESIAN_POINT('',(3.3,0.5,4.3));
#5285=CARTESIAN_POINT('',(3.3,-0.5,4.3));
#5286=CARTESIAN_POINT('Origin',(-3.3,-0.5,4.3));
#5287=CARTESIAN_POINT('',(-3.3,-0.5,4.3));
#5288=CARTESIAN_POINT('',(-3.3,-0.5,4.3));
#5289=CARTESIAN_POINT('',(-3.3,0.5,4.3));
#5290=CARTESIAN_POINT('',(-3.3,0.5,4.3));
#5291=CARTESIAN_POINT('',(-3.3,-0.5,4.3));
#5292=CARTESIAN_POINT('Origin',(-4.3,-0.5,3.3));
#5293=CARTESIAN_POINT('',(-4.3,-0.5,3.3));
#5294=CARTESIAN_POINT('',(-4.3,0.5,3.3));
#5295=CARTESIAN_POINT('Origin',(0.,0.5,0.));
#5296=CARTESIAN_POINT('Origin',(0.,-0.5,0.));
#6768=UNCERTAINTY_MEASURE_WITH_UNIT(LENGTH_MEASURE(0.001),#6806,
'DISTANCE_ACCURACY_VALUE',
'Maximum model space distance between geometric entities at asserted c
onnectivities');
#6780=UNCERTAINTY_MEASURE_WITH_UNIT(LENGTH_MEASURE(0.001),#6806,
'DISTANCE_ACCURACY_VALUE',
'Maximum model space distance between geometric entities at asserted c
onnectivities');
#6793=(
GEOMETRIC_REPRESENTATION_CONTEXT(3)
GLOBAL_UNCERTAINTY_ASSIGNED_CONTEXT((#6768))
GLOBAL_UNIT_ASSIGNED_CONTEXT((#6806,#6808,#6809))
REPRESENTATION_CONTEXT('','3D')
);
#6805=(
GEOMETRIC_REPRESENTATION_CONTEXT(3)
GLOBAL_UNCERTAINTY_ASSIGNED_CONTEXT((#6780))
GLOBAL_UNIT_ASSIGNED_CONTEXT((#6806,#6808,#6809))
REPRESENTATION_CONTEXT('','3D')
);
#6806=(
LENGTH_UNIT()
NAMED_UNIT(*)
SI_UNIT(.CENTI.,.METRE.)
);
#6808=(
NAMED_UNIT(*)
PLANE_ANGLE_UNIT()
SI_UNIT($,.RADIAN.)
);
#6809=(
NAMED_UNIT(*)
SI_UNIT($,.STERADIAN.)
SOLID_ANGLE_UNIT()
);
#6822=SHAPE_DEFINITION_REPRESENTATION(#6846,#6910);
#6846=PRODUCT_DEFINITION_SHAPE('',$,#6935);
#6910=SHAPE_REPRESENTATION('',(#3674),#6793);
#6922=PRODUCT_DEFINITION_CONTEXT('part definition',#6996,'design');
#6935=PRODUCT_DEFINITION('Housing','Housing',#6959,#6922);
#6959=PRODUCT_DEFINITION_FORMATION('',$,#7010);
#6996=APPLICATION_CONTEXT(
'Core Data for Automotive Mechanical Design Process');
#6997=PRODUCT_CONTEXT('part definition',#6996,'mechanical');
#7010=PRODUCT('Housing','Housing','Housing',(#6997));
#7064=COLOUR_RGB('Dark Blue',0.08,0.2,0.34);
#7065=FILL_AREA_STYLE_COLOUR('',#7064);
#7066=FILL_AREA_STYLE('',(#7065));
#7067=SURFACE_STYLE_FILL_AREA(#7066);
#7068=SURFACE_SIDE_STYLE('',(#7067));
#7069=SURFACE_STYLE_USAGE(.BOTH.,#7068);
#7070=PRESENTATION_STYLE_ASSIGNMENT((#7069));
ENDSEC;
END-ISO-10303-21;
